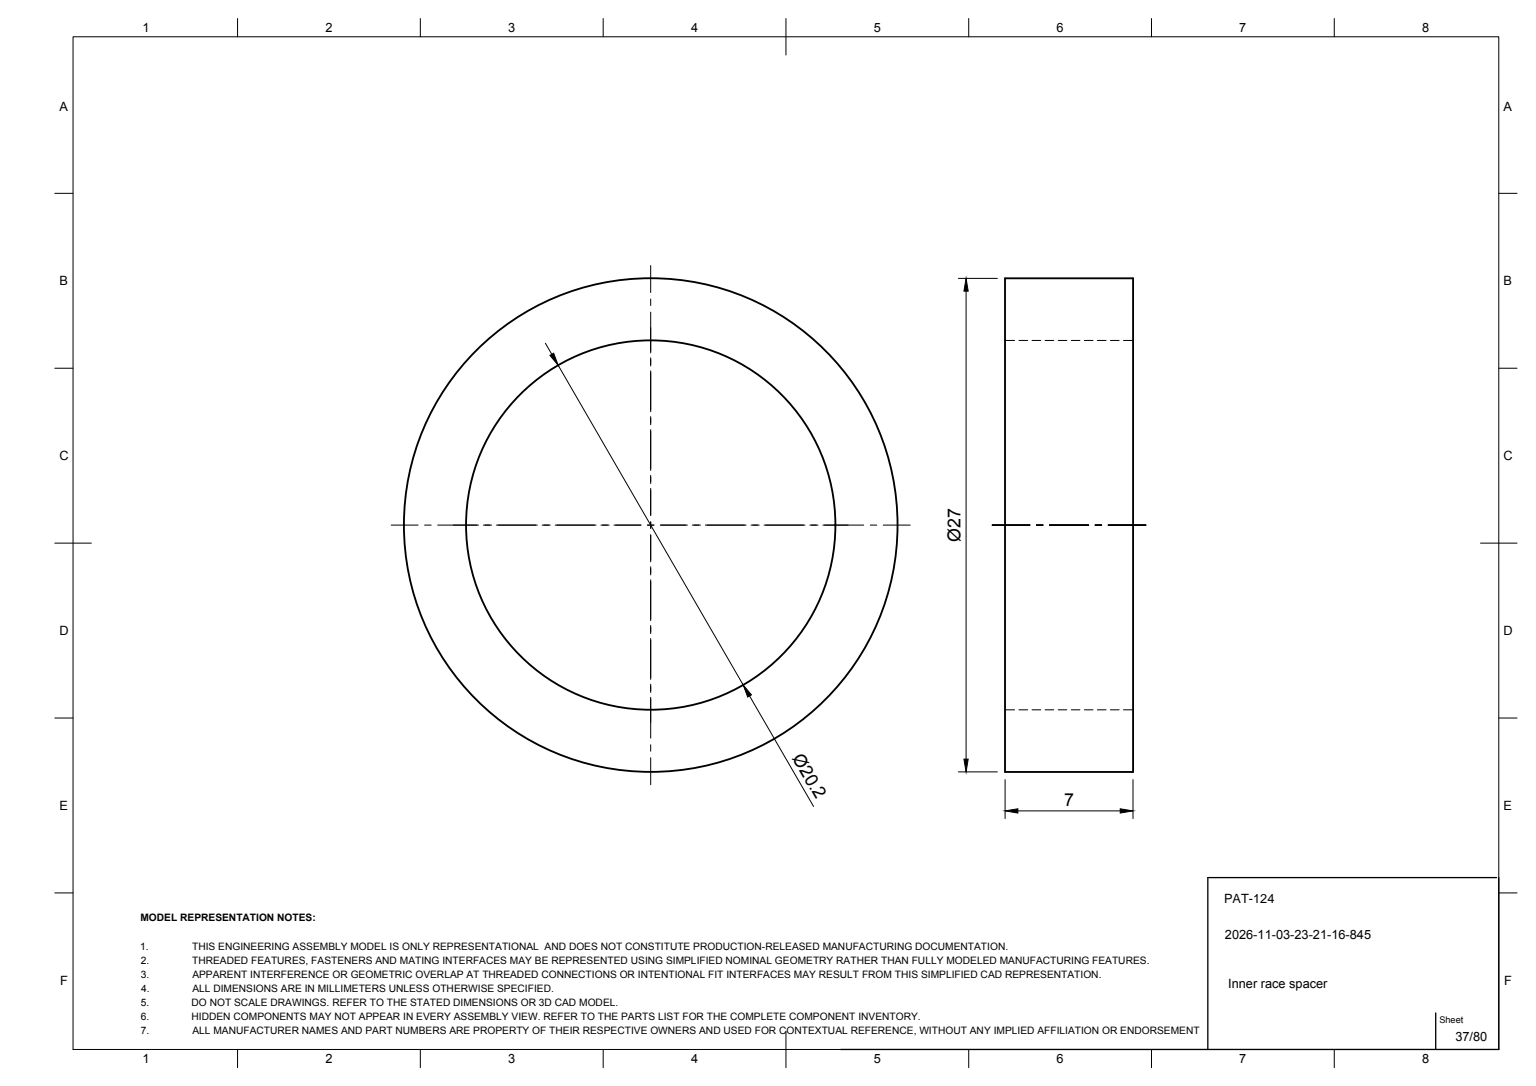
ISO-10303-21;
HEADER;
/* Generated by software containing ST-Developer
 * from STEP Tools, Inc. (www.steptools.com) 
 */

FILE_DESCRIPTION(
/* description */ ('XY cross-slide table'),
/* implementation_level */ '2;1');

FILE_NAME(
/* name */ 'Inner race spacer.step',
/* time_stamp */ '2026-10-28T03:22:46-07:00',
/* author */ (''),
/* organization */ (''),
/* preprocessor_version */ 'ST-DEVELOPER v20.2',
/* originating_system */ 'Autodesk Translation Framework v15.17.0.0',
/* authorisation */ '');

FILE_SCHEMA (('AUTOMOTIVE_DESIGN { 1 0 10303 214 3 1 1 }'));
ENDSEC;

DATA;
#10=MECHANICAL_DESIGN_GEOMETRIC_PRESENTATION_REPRESENTATION('',(#1718),#62984);
#1537=SHAPE_REPRESENTATION_RELATIONSHIP('SRR','None',#63390,#1620);
#1620=ADVANCED_BREP_SHAPE_REPRESENTATION('',(#1828),#62927);
#1718=STYLED_ITEM('',(#63912),#1828);
#1828=MANIFOLD_SOLID_BREP('Body1',#23015);
#2065=FACE_BOUND('',#4932,.T.);
#2066=FACE_BOUND('',#4934,.T.);
#2527=PLANE('',#25032);
#2528=PLANE('',#25033);
#3437=FACE_OUTER_BOUND('',#4929,.T.);
#3438=FACE_OUTER_BOUND('',#4930,.T.);
#3439=FACE_OUTER_BOUND('',#4931,.T.);
#3440=FACE_OUTER_BOUND('',#4933,.T.);
#4929=EDGE_LOOP('',(#17620,#17621,#17622,#17623));
#4930=EDGE_LOOP('',(#17624,#17625,#17626,#17627));
#4931=EDGE_LOOP('',(#17628));
#4932=EDGE_LOOP('',(#17629));
#4933=EDGE_LOOP('',(#17630));
#4934=EDGE_LOOP('',(#17631));
#6543=LINE('',#47282,#8030);
#6544=LINE('',#47288,#8031);
#8030=VECTOR('',#29154,1.01);
#8031=VECTOR('',#29161,1.35);
#9267=CIRCLE('',#25027,1.01);
#9268=CIRCLE('',#25028,1.01);
#9269=CIRCLE('',#25030,1.35);
#9270=CIRCLE('',#25031,1.35);
#10689=VERTEX_POINT('',#47279);
#10690=VERTEX_POINT('',#47281);
#10691=VERTEX_POINT('',#47285);
#10692=VERTEX_POINT('',#47287);
#13194=EDGE_CURVE('',#10689,#10689,#9267,.T.);
#13195=EDGE_CURVE('',#10689,#10690,#6543,.T.);
#13196=EDGE_CURVE('',#10690,#10690,#9268,.T.);
#13197=EDGE_CURVE('',#10691,#10691,#9269,.T.);
#13198=EDGE_CURVE('',#10691,#10692,#6544,.T.);
#13199=EDGE_CURVE('',#10692,#10692,#9270,.T.);
#17620=ORIENTED_EDGE('',*,*,#13194,.F.);
#17621=ORIENTED_EDGE('',*,*,#13195,.T.);
#17622=ORIENTED_EDGE('',*,*,#13196,.T.);
#17623=ORIENTED_EDGE('',*,*,#13195,.F.);
#17624=ORIENTED_EDGE('',*,*,#13197,.F.);
#17625=ORIENTED_EDGE('',*,*,#13198,.T.);
#17626=ORIENTED_EDGE('',*,*,#13199,.T.);
#17627=ORIENTED_EDGE('',*,*,#13198,.F.);
#17628=ORIENTED_EDGE('',*,*,#13197,.T.);
#17629=ORIENTED_EDGE('',*,*,#13194,.T.);
#17630=ORIENTED_EDGE('',*,*,#13199,.F.);
#17631=ORIENTED_EDGE('',*,*,#13196,.F.);
#21319=CYLINDRICAL_SURFACE('',#25026,1.01);
#21320=CYLINDRICAL_SURFACE('',#25029,1.35);
#22218=ADVANCED_FACE('',(#3437),#21319,.F.);
#22219=ADVANCED_FACE('',(#3438),#21320,.T.);
#22220=ADVANCED_FACE('',(#3439,#2065),#2527,.T.);
#22221=ADVANCED_FACE('',(#3440,#2066),#2528,.F.);
#23015=CLOSED_SHELL('',(#22218,#22219,#22220,#22221));
#25025=AXIS2_PLACEMENT_3D('',#47277,#29148,#29149);
#25026=AXIS2_PLACEMENT_3D('',#47278,#29150,#29151);
#25027=AXIS2_PLACEMENT_3D('',#47280,#29152,#29153);
#25028=AXIS2_PLACEMENT_3D('',#47283,#29155,#29156);
#25029=AXIS2_PLACEMENT_3D('',#47284,#29157,#29158);
#25030=AXIS2_PLACEMENT_3D('',#47286,#29159,#29160);
#25031=AXIS2_PLACEMENT_3D('',#47289,#29162,#29163);
#25032=AXIS2_PLACEMENT_3D('',#47290,#29164,#29165);
#25033=AXIS2_PLACEMENT_3D('',#47291,#29166,#29167);
#29148=DIRECTION('axis',(0.,0.,1.));
#29149=DIRECTION('refdir',(1.,0.,0.));
#29150=DIRECTION('center_axis',(1.,0.,0.));
#29151=DIRECTION('ref_axis',(0.,0.,-1.));
#29152=DIRECTION('center_axis',(-1.,0.,0.));
#29153=DIRECTION('ref_axis',(0.,0.,-1.));
#29154=DIRECTION('',(-1.,0.,0.));
#29155=DIRECTION('center_axis',(-1.,0.,0.));
#29156=DIRECTION('ref_axis',(0.,0.,-1.));
#29157=DIRECTION('center_axis',(1.,0.,0.));
#29158=DIRECTION('ref_axis',(0.,0.,-1.));
#29159=DIRECTION('center_axis',(1.,0.,0.));
#29160=DIRECTION('ref_axis',(0.,0.,-1.));
#29161=DIRECTION('',(-1.,0.,0.));
#29162=DIRECTION('center_axis',(1.,0.,0.));
#29163=DIRECTION('ref_axis',(0.,0.,-1.));
#29164=DIRECTION('center_axis',(1.,0.,0.));
#29165=DIRECTION('ref_axis',(0.,0.,-1.));
#29166=DIRECTION('center_axis',(1.,0.,0.));
#29167=DIRECTION('ref_axis',(0.,0.,-1.));
#47277=CARTESIAN_POINT('',(0.,0.,0.));
#47278=CARTESIAN_POINT('Origin',(24.7,0.,4.));
#47279=CARTESIAN_POINT('',(25.4,-1.23689326713883E-16,5.01));
#47280=CARTESIAN_POINT('Origin',(25.4,0.,4.));
#47281=CARTESIAN_POINT('',(24.7,-1.23689326713883E-16,5.01));
#47282=CARTESIAN_POINT('',(24.7,-1.23689326713883E-16,5.01));
#47283=CARTESIAN_POINT('Origin',(24.7,0.,4.));
#47284=CARTESIAN_POINT('Origin',(24.7,0.,4.));
#47285=CARTESIAN_POINT('',(25.4,-1.65327317884893E-16,5.35));
#47286=CARTESIAN_POINT('Origin',(25.4,0.,4.));
#47287=CARTESIAN_POINT('',(24.7,-1.65327317884893E-16,5.35));
#47288=CARTESIAN_POINT('',(24.7,-1.65327317884893E-16,5.35));
#47289=CARTESIAN_POINT('Origin',(24.7,0.,4.));
#47290=CARTESIAN_POINT('Origin',(25.4,0.,4.));
#47291=CARTESIAN_POINT('Origin',(24.7,0.,4.));
#62828=UNCERTAINTY_MEASURE_WITH_UNIT(LENGTH_MEASURE(0.001),#62985,
'DISTANCE_ACCURACY_VALUE',
'Maximum model space distance between geometric entities at asserted c
onnectivities');
#62885=UNCERTAINTY_MEASURE_WITH_UNIT(LENGTH_MEASURE(0.001),#62985,
'DISTANCE_ACCURACY_VALUE',
'Maximum model space distance between geometric entities at asserted c
onnectivities');
#62927=(
GEOMETRIC_REPRESENTATION_CONTEXT(3)
GLOBAL_UNCERTAINTY_ASSIGNED_CONTEXT((#62828))
GLOBAL_UNIT_ASSIGNED_CONTEXT((#62985,#62987,#62988))
REPRESENTATION_CONTEXT('','3D')
);
#62984=(
GEOMETRIC_REPRESENTATION_CONTEXT(3)
GLOBAL_UNCERTAINTY_ASSIGNED_CONTEXT((#62885))
GLOBAL_UNIT_ASSIGNED_CONTEXT((#62985,#62987,#62988))
REPRESENTATION_CONTEXT('','3D')
);
#62985=(
LENGTH_UNIT()
NAMED_UNIT(*)
SI_UNIT(.CENTI.,.METRE.)
);
#62987=(
NAMED_UNIT(*)
PLANE_ANGLE_UNIT()
SI_UNIT($,.RADIAN.)
);
#62988=(
NAMED_UNIT(*)
SI_UNIT($,.STERADIAN.)
SOLID_ANGLE_UNIT()
);
#63030=SHAPE_DEFINITION_REPRESENTATION(#63161,#63390);
#63161=PRODUCT_DEFINITION_SHAPE('',$,#63489);
#63390=SHAPE_REPRESENTATION('',(#25025),#62927);
#63447=PRODUCT_DEFINITION_CONTEXT('part definition',#63743,'design');
#63489=PRODUCT_DEFINITION('Inner race spacer','Inner race spacer',#63587,
#63447);
#63587=PRODUCT_DEFINITION_FORMATION('',$,#63786);
#63743=APPLICATION_CONTEXT(
'Core Data for Automotive Mechanical Design Process');
#63744=PRODUCT_CONTEXT('part definition',#63743,'mechanical');
#63786=PRODUCT('Inner race spacer','Inner race spacer',
'Inner race spacer',(#63744));
#63906=COLOUR_RGB('Grey',0.48,0.52,0.57);
#63907=FILL_AREA_STYLE_COLOUR('',#63906);
#63908=FILL_AREA_STYLE('',(#63907));
#63909=SURFACE_STYLE_FILL_AREA(#63908);
#63910=SURFACE_SIDE_STYLE('',(#63909));
#63911=SURFACE_STYLE_USAGE(.BOTH.,#63910);
#63912=PRESENTATION_STYLE_ASSIGNMENT((#63911));
ENDSEC;
END-ISO-10303-21;
